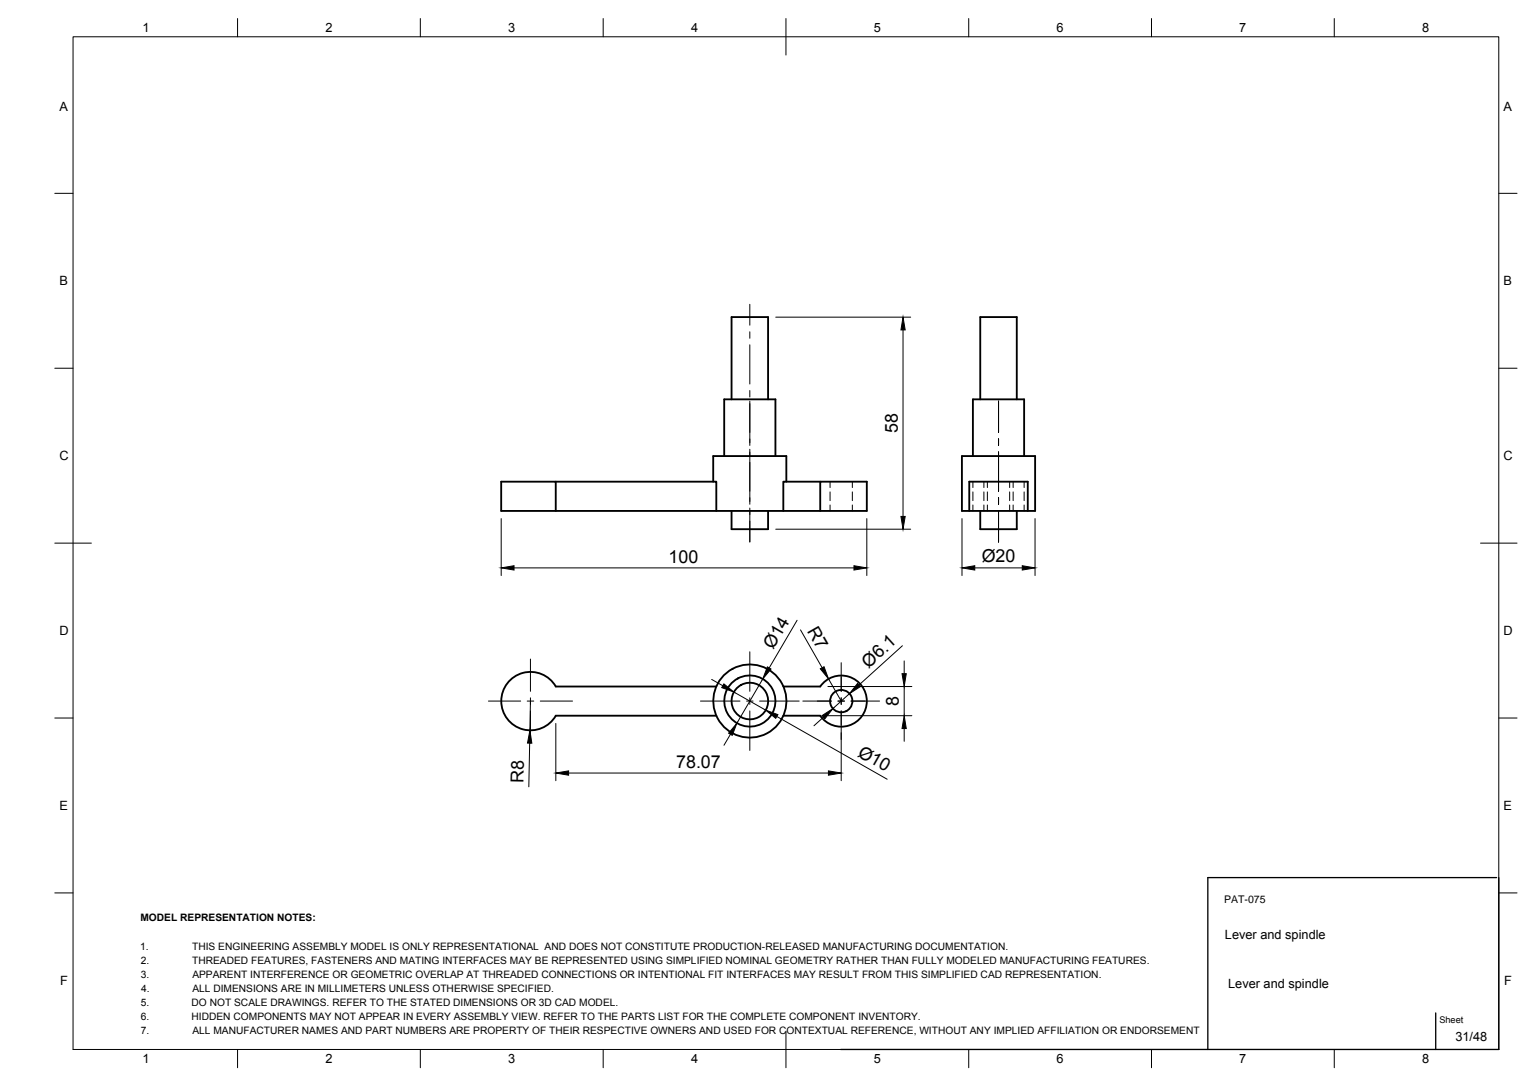
ISO-10303-21;
HEADER;
/* Generated by software containing ST-Developer
 * from STEP Tools, Inc. (www.steptools.com) 
 */

FILE_DESCRIPTION(
/* description */ ('Over-Centre Plunger Toggle Clamp on Slotted Fixture Frame'),
/* implementation_level */ '2;1');

FILE_NAME(
/* name */ 
'Lever and spindle.step',
/* time_stamp */ '2026-10-28T03:23:24-07:00',
/* author */ (''),
/* organization */ (''),
/* preprocessor_version */ 'ST-DEVELOPER v20.2',
/* originating_system */ 'Autodesk Translation Framework v15.17.0.0',
/* authorisation */ '');

FILE_SCHEMA (('AUTOMOTIVE_DESIGN { 1 0 10303 214 3 1 1 }'));
ENDSEC;

DATA;
#10=MECHANICAL_DESIGN_GEOMETRIC_PRESENTATION_REPRESENTATION('',(#545),#15212);
#453=SHAPE_REPRESENTATION_RELATIONSHIP('SRR','None',#15430,#495);
#495=ADVANCED_BREP_SHAPE_REPRESENTATION('',(#594),#15192);
#545=STYLED_ITEM('',(#15712),#594);
#594=MANIFOLD_SOLID_BREP('Body1',#8279);
#742=FACE_BOUND('',#2033,.T.);
#743=FACE_BOUND('',#2034,.T.);
#744=FACE_BOUND('',#2041,.T.);
#745=FACE_BOUND('',#2044,.T.);
#746=FACE_BOUND('',#2047,.T.);
#984=PLANE('',#9388);
#985=PLANE('',#9394);
#986=PLANE('',#9395);
#987=PLANE('',#9397);
#988=PLANE('',#9400);
#989=PLANE('',#9401);
#990=PLANE('',#9403);
#991=PLANE('',#9404);
#992=PLANE('',#9408);
#993=PLANE('',#9416);
#994=PLANE('',#9417);
#1413=FACE_OUTER_BOUND('',#2030,.T.);
#1414=FACE_OUTER_BOUND('',#2031,.T.);
#1415=FACE_OUTER_BOUND('',#2032,.T.);
#1416=FACE_OUTER_BOUND('',#2035,.T.);
#1417=FACE_OUTER_BOUND('',#2036,.T.);
#1418=FACE_OUTER_BOUND('',#2037,.T.);
#1419=FACE_OUTER_BOUND('',#2038,.T.);
#1420=FACE_OUTER_BOUND('',#2039,.T.);
#1421=FACE_OUTER_BOUND('',#2040,.T.);
#1422=FACE_OUTER_BOUND('',#2042,.T.);
#1423=FACE_OUTER_BOUND('',#2043,.T.);
#1424=FACE_OUTER_BOUND('',#2045,.T.);
#1425=FACE_OUTER_BOUND('',#2046,.T.);
#1426=FACE_OUTER_BOUND('',#2048,.T.);
#1427=FACE_OUTER_BOUND('',#2049,.T.);
#1428=FACE_OUTER_BOUND('',#2050,.T.);
#1429=FACE_OUTER_BOUND('',#2051,.T.);
#1430=FACE_OUTER_BOUND('',#2052,.T.);
#2030=EDGE_LOOP('',(#7007,#7008,#7009,#7010));
#2031=EDGE_LOOP('',(#7011,#7012,#7013,#7014));
#2032=EDGE_LOOP('',(#7015,#7016,#7017,#7018,#7019,#7020,#7021,#7022,#7023));
#2033=EDGE_LOOP('',(#7024));
#2034=EDGE_LOOP('',(#7025));
#2035=EDGE_LOOP('',(#7026,#7027,#7028,#7029));
#2036=EDGE_LOOP('',(#7030,#7031,#7032,#7033));
#2037=EDGE_LOOP('',(#7034,#7035,#7036,#7037));
#2038=EDGE_LOOP('',(#7038,#7039,#7040,#7041));
#2039=EDGE_LOOP('',(#7042,#7043,#7044,#7045));
#2040=EDGE_LOOP('',(#7046,#7047,#7048,#7049));
#2041=EDGE_LOOP('',(#7050));
#2042=EDGE_LOOP('',(#7051,#7052,#7053,#7054));
#2043=EDGE_LOOP('',(#7055));
#2044=EDGE_LOOP('',(#7056));
#2045=EDGE_LOOP('',(#7057,#7058,#7059,#7060,#7061,#7062,#7063,#7064,#7065,
#7066,#7067,#7068));
#2046=EDGE_LOOP('',(#7069));
#2047=EDGE_LOOP('',(#7070));
#2048=EDGE_LOOP('',(#7071,#7072,#7073,#7074));
#2049=EDGE_LOOP('',(#7075,#7076,#7077,#7078));
#2050=EDGE_LOOP('',(#7079,#7080,#7081,#7082));
#2051=EDGE_LOOP('',(#7083));
#2052=EDGE_LOOP('',(#7084));
#2676=LINE('',#14276,#3306);
#2677=LINE('',#14281,#3307);
#2678=LINE('',#14285,#3308);
#2679=LINE('',#14289,#3309);
#2680=LINE('',#14295,#3310);
#2681=LINE('',#14299,#3311);
#2682=LINE('',#14302,#3312);
#2683=LINE('',#14307,#3313);
#2684=LINE('',#14308,#3314);
#2685=LINE('',#14311,#3315);
#2686=LINE('',#14314,#3316);
#2687=LINE('',#14317,#3317);
#2688=LINE('',#14320,#3318);
#2689=LINE('',#14323,#3319);
#2690=LINE('',#14324,#3320);
#2691=LINE('',#14327,#3321);
#2692=LINE('',#14330,#3322);
#2693=LINE('',#14337,#3323);
#2694=LINE('',#14344,#3324);
#2695=LINE('',#14347,#3325);
#2696=LINE('',#14352,#3326);
#3306=VECTOR('',#11441,0.305);
#3307=VECTOR('',#11446,1.);
#3308=VECTOR('',#11449,1.);
#3309=VECTOR('',#11454,1.);
#3310=VECTOR('',#11459,1.);
#3311=VECTOR('',#11462,1.);
#3312=VECTOR('',#11465,1.);
#3313=VECTOR('',#11470,1.);
#3314=VECTOR('',#11471,1.);
#3315=VECTOR('',#11474,1.);
#3316=VECTOR('',#11479,1.);
#3317=VECTOR('',#11482,1.);
#3318=VECTOR('',#11485,1.);
#3319=VECTOR('',#11488,1.);
#3320=VECTOR('',#11489,1.);
#3321=VECTOR('',#11492,1.);
#3322=VECTOR('',#11497,1.);
#3323=VECTOR('',#11506,1.);
#3324=VECTOR('',#11515,0.7);
#3325=VECTOR('',#11518,0.5);
#3326=VECTOR('',#11525,0.5);
#3745=CIRCLE('',#9383,0.305);
#3746=CIRCLE('',#9384,0.305);
#3747=CIRCLE('',#9386,0.8);
#3748=CIRCLE('',#9387,0.8);
#3749=CIRCLE('',#9389,1.);
#3750=CIRCLE('',#9390,1.);
#3751=CIRCLE('',#9391,0.7);
#3752=CIRCLE('',#9392,1.);
#3753=CIRCLE('',#9393,0.5);
#3754=CIRCLE('',#9396,1.);
#3755=CIRCLE('',#9399,0.7);
#3756=CIRCLE('',#9402,1.);
#3757=CIRCLE('',#9405,1.);
#3758=CIRCLE('',#9406,0.7);
#3759=CIRCLE('',#9409,0.7);
#3760=CIRCLE('',#9410,0.5);
#3761=CIRCLE('',#9413,0.5);
#3762=CIRCLE('',#9415,0.5);
#4345=VERTEX_POINT('',#14273);
#4346=VERTEX_POINT('',#14275);
#4347=VERTEX_POINT('',#14279);
#4348=VERTEX_POINT('',#14280);
#4349=VERTEX_POINT('',#14282);
#4350=VERTEX_POINT('',#14284);
#4351=VERTEX_POINT('',#14288);
#4352=VERTEX_POINT('',#14290);
#4353=VERTEX_POINT('',#14292);
#4354=VERTEX_POINT('',#14294);
#4355=VERTEX_POINT('',#14296);
#4356=VERTEX_POINT('',#14298);
#4357=VERTEX_POINT('',#14300);
#4358=VERTEX_POINT('',#14303);
#4359=VERTEX_POINT('',#14306);
#4360=VERTEX_POINT('',#14310);
#4361=VERTEX_POINT('',#14316);
#4362=VERTEX_POINT('',#14318);
#4363=VERTEX_POINT('',#14322);
#4364=VERTEX_POINT('',#14326);
#4365=VERTEX_POINT('',#14332);
#4366=VERTEX_POINT('',#14334);
#4367=VERTEX_POINT('',#14339);
#4368=VERTEX_POINT('',#14341);
#4369=VERTEX_POINT('',#14346);
#4370=VERTEX_POINT('',#14350);
#5264=EDGE_CURVE('',#4345,#4345,#3745,.T.);
#5265=EDGE_CURVE('',#4345,#4346,#2676,.T.);
#5266=EDGE_CURVE('',#4346,#4346,#3746,.T.);
#5267=EDGE_CURVE('',#4347,#4348,#2677,.T.);
#5268=EDGE_CURVE('',#4349,#4347,#3747,.T.);
#5269=EDGE_CURVE('',#4350,#4349,#2678,.T.);
#5270=EDGE_CURVE('',#4350,#4348,#3748,.T.);
#5271=EDGE_CURVE('',#4351,#4350,#2679,.T.);
#5272=EDGE_CURVE('',#4352,#4351,#3749,.T.);
#5273=EDGE_CURVE('',#4353,#4352,#3750,.T.);
#5274=EDGE_CURVE('',#4354,#4353,#2680,.T.);
#5275=EDGE_CURVE('',#4355,#4354,#3751,.T.);
#5276=EDGE_CURVE('',#4356,#4355,#2681,.T.);
#5277=EDGE_CURVE('',#4357,#4356,#3752,.T.);
#5278=EDGE_CURVE('',#4348,#4357,#2682,.T.);
#5279=EDGE_CURVE('',#4358,#4358,#3753,.T.);
#5280=EDGE_CURVE('',#4359,#4349,#2683,.T.);
#5281=EDGE_CURVE('',#4351,#4359,#2684,.T.);
#5282=EDGE_CURVE('',#4347,#4360,#2685,.T.);
#5283=EDGE_CURVE('',#4359,#4360,#3754,.T.);
#5284=EDGE_CURVE('',#4360,#4357,#2686,.T.);
#5285=EDGE_CURVE('',#4361,#4354,#2687,.T.);
#5286=EDGE_CURVE('',#4362,#4361,#3755,.T.);
#5287=EDGE_CURVE('',#4355,#4362,#2688,.T.);
#5288=EDGE_CURVE('',#4363,#4362,#2689,.T.);
#5289=EDGE_CURVE('',#4356,#4363,#2690,.T.);
#5290=EDGE_CURVE('',#4361,#4364,#2691,.T.);
#5291=EDGE_CURVE('',#4363,#4364,#3756,.T.);
#5292=EDGE_CURVE('',#4364,#4353,#2692,.T.);
#5293=EDGE_CURVE('',#4365,#4365,#3757,.T.);
#5294=EDGE_CURVE('',#4366,#4366,#3758,.T.);
#5295=EDGE_CURVE('',#4365,#4352,#2693,.T.);
#5296=EDGE_CURVE('',#4367,#4367,#3759,.T.);
#5297=EDGE_CURVE('',#4368,#4368,#3760,.T.);
#5298=EDGE_CURVE('',#4367,#4366,#2694,.T.);
#5299=EDGE_CURVE('',#4358,#4369,#2695,.T.);
#5300=EDGE_CURVE('',#4369,#4369,#3761,.T.);
#5301=EDGE_CURVE('',#4370,#4370,#3762,.T.);
#5302=EDGE_CURVE('',#4370,#4368,#2696,.T.);
#7007=ORIENTED_EDGE('',*,*,#5264,.F.);
#7008=ORIENTED_EDGE('',*,*,#5265,.T.);
#7009=ORIENTED_EDGE('',*,*,#5266,.F.);
#7010=ORIENTED_EDGE('',*,*,#5265,.F.);
#7011=ORIENTED_EDGE('',*,*,#5267,.F.);
#7012=ORIENTED_EDGE('',*,*,#5268,.F.);
#7013=ORIENTED_EDGE('',*,*,#5269,.F.);
#7014=ORIENTED_EDGE('',*,*,#5270,.T.);
#7015=ORIENTED_EDGE('',*,*,#5270,.F.);
#7016=ORIENTED_EDGE('',*,*,#5271,.F.);
#7017=ORIENTED_EDGE('',*,*,#5272,.F.);
#7018=ORIENTED_EDGE('',*,*,#5273,.F.);
#7019=ORIENTED_EDGE('',*,*,#5274,.F.);
#7020=ORIENTED_EDGE('',*,*,#5275,.F.);
#7021=ORIENTED_EDGE('',*,*,#5276,.F.);
#7022=ORIENTED_EDGE('',*,*,#5277,.F.);
#7023=ORIENTED_EDGE('',*,*,#5278,.F.);
#7024=ORIENTED_EDGE('',*,*,#5264,.T.);
#7025=ORIENTED_EDGE('',*,*,#5279,.F.);
#7026=ORIENTED_EDGE('',*,*,#5269,.T.);
#7027=ORIENTED_EDGE('',*,*,#5280,.F.);
#7028=ORIENTED_EDGE('',*,*,#5281,.F.);
#7029=ORIENTED_EDGE('',*,*,#5271,.T.);
#7030=ORIENTED_EDGE('',*,*,#5282,.T.);
#7031=ORIENTED_EDGE('',*,*,#5283,.F.);
#7032=ORIENTED_EDGE('',*,*,#5280,.T.);
#7033=ORIENTED_EDGE('',*,*,#5268,.T.);
#7034=ORIENTED_EDGE('',*,*,#5267,.T.);
#7035=ORIENTED_EDGE('',*,*,#5278,.T.);
#7036=ORIENTED_EDGE('',*,*,#5284,.F.);
#7037=ORIENTED_EDGE('',*,*,#5282,.F.);
#7038=ORIENTED_EDGE('',*,*,#5285,.F.);
#7039=ORIENTED_EDGE('',*,*,#5286,.F.);
#7040=ORIENTED_EDGE('',*,*,#5287,.F.);
#7041=ORIENTED_EDGE('',*,*,#5275,.T.);
#7042=ORIENTED_EDGE('',*,*,#5287,.T.);
#7043=ORIENTED_EDGE('',*,*,#5288,.F.);
#7044=ORIENTED_EDGE('',*,*,#5289,.F.);
#7045=ORIENTED_EDGE('',*,*,#5276,.T.);
#7046=ORIENTED_EDGE('',*,*,#5290,.T.);
#7047=ORIENTED_EDGE('',*,*,#5291,.F.);
#7048=ORIENTED_EDGE('',*,*,#5288,.T.);
#7049=ORIENTED_EDGE('',*,*,#5286,.T.);
#7050=ORIENTED_EDGE('',*,*,#5266,.T.);
#7051=ORIENTED_EDGE('',*,*,#5285,.T.);
#7052=ORIENTED_EDGE('',*,*,#5274,.T.);
#7053=ORIENTED_EDGE('',*,*,#5292,.F.);
#7054=ORIENTED_EDGE('',*,*,#5290,.F.);
#7055=ORIENTED_EDGE('',*,*,#5293,.T.);
#7056=ORIENTED_EDGE('',*,*,#5294,.F.);
#7057=ORIENTED_EDGE('',*,*,#5293,.F.);
#7058=ORIENTED_EDGE('',*,*,#5295,.T.);
#7059=ORIENTED_EDGE('',*,*,#5272,.T.);
#7060=ORIENTED_EDGE('',*,*,#5281,.T.);
#7061=ORIENTED_EDGE('',*,*,#5283,.T.);
#7062=ORIENTED_EDGE('',*,*,#5284,.T.);
#7063=ORIENTED_EDGE('',*,*,#5277,.T.);
#7064=ORIENTED_EDGE('',*,*,#5289,.T.);
#7065=ORIENTED_EDGE('',*,*,#5291,.T.);
#7066=ORIENTED_EDGE('',*,*,#5292,.T.);
#7067=ORIENTED_EDGE('',*,*,#5273,.T.);
#7068=ORIENTED_EDGE('',*,*,#5295,.F.);
#7069=ORIENTED_EDGE('',*,*,#5296,.T.);
#7070=ORIENTED_EDGE('',*,*,#5297,.F.);
#7071=ORIENTED_EDGE('',*,*,#5296,.F.);
#7072=ORIENTED_EDGE('',*,*,#5298,.T.);
#7073=ORIENTED_EDGE('',*,*,#5294,.T.);
#7074=ORIENTED_EDGE('',*,*,#5298,.F.);
#7075=ORIENTED_EDGE('',*,*,#5279,.T.);
#7076=ORIENTED_EDGE('',*,*,#5299,.T.);
#7077=ORIENTED_EDGE('',*,*,#5300,.T.);
#7078=ORIENTED_EDGE('',*,*,#5299,.F.);
#7079=ORIENTED_EDGE('',*,*,#5301,.F.);
#7080=ORIENTED_EDGE('',*,*,#5302,.T.);
#7081=ORIENTED_EDGE('',*,*,#5297,.T.);
#7082=ORIENTED_EDGE('',*,*,#5302,.F.);
#7083=ORIENTED_EDGE('',*,*,#5301,.T.);
#7084=ORIENTED_EDGE('',*,*,#5300,.F.);
#7712=CYLINDRICAL_SURFACE('',#9382,0.305);
#7713=CYLINDRICAL_SURFACE('',#9385,0.8);
#7714=CYLINDRICAL_SURFACE('',#9398,0.7);
#7715=CYLINDRICAL_SURFACE('',#9407,1.);
#7716=CYLINDRICAL_SURFACE('',#9411,0.7);
#7717=CYLINDRICAL_SURFACE('',#9412,0.5);
#7718=CYLINDRICAL_SURFACE('',#9414,0.5);
#8085=ADVANCED_FACE('',(#1413),#7712,.F.);
#8086=ADVANCED_FACE('',(#1414),#7713,.T.);
#8087=ADVANCED_FACE('',(#1415,#742,#743),#984,.F.);
#8088=ADVANCED_FACE('',(#1416),#985,.T.);
#8089=ADVANCED_FACE('',(#1417),#986,.T.);
#8090=ADVANCED_FACE('',(#1418),#987,.T.);
#8091=ADVANCED_FACE('',(#1419),#7714,.T.);
#8092=ADVANCED_FACE('',(#1420),#988,.T.);
#8093=ADVANCED_FACE('',(#1421,#744),#989,.T.);
#8094=ADVANCED_FACE('',(#1422),#990,.T.);
#8095=ADVANCED_FACE('',(#1423,#745),#991,.T.);
#8096=ADVANCED_FACE('',(#1424),#7715,.T.);
#8097=ADVANCED_FACE('',(#1425,#746),#992,.T.);
#8098=ADVANCED_FACE('',(#1426),#7716,.T.);
#8099=ADVANCED_FACE('',(#1427),#7717,.T.);
#8100=ADVANCED_FACE('',(#1428),#7718,.T.);
#8101=ADVANCED_FACE('',(#1429),#993,.T.);
#8102=ADVANCED_FACE('',(#1430),#994,.F.);
#8279=CLOSED_SHELL('',(#8085,#8086,#8087,#8088,#8089,#8090,#8091,#8092,
#8093,#8094,#8095,#8096,#8097,#8098,#8099,#8100,#8101,#8102));
#9381=AXIS2_PLACEMENT_3D('',#14271,#11435,#11436);
#9382=AXIS2_PLACEMENT_3D('',#14272,#11437,#11438);
#9383=AXIS2_PLACEMENT_3D('',#14274,#11439,#11440);
#9384=AXIS2_PLACEMENT_3D('',#14277,#11442,#11443);
#9385=AXIS2_PLACEMENT_3D('',#14278,#11444,#11445);
#9386=AXIS2_PLACEMENT_3D('',#14283,#11447,#11448);
#9387=AXIS2_PLACEMENT_3D('',#14286,#11450,#11451);
#9388=AXIS2_PLACEMENT_3D('',#14287,#11452,#11453);
#9389=AXIS2_PLACEMENT_3D('',#14291,#11455,#11456);
#9390=AXIS2_PLACEMENT_3D('',#14293,#11457,#11458);
#9391=AXIS2_PLACEMENT_3D('',#14297,#11460,#11461);
#9392=AXIS2_PLACEMENT_3D('',#14301,#11463,#11464);
#9393=AXIS2_PLACEMENT_3D('',#14304,#11466,#11467);
#9394=AXIS2_PLACEMENT_3D('',#14305,#11468,#11469);
#9395=AXIS2_PLACEMENT_3D('',#14309,#11472,#11473);
#9396=AXIS2_PLACEMENT_3D('',#14312,#11475,#11476);
#9397=AXIS2_PLACEMENT_3D('',#14313,#11477,#11478);
#9398=AXIS2_PLACEMENT_3D('',#14315,#11480,#11481);
#9399=AXIS2_PLACEMENT_3D('',#14319,#11483,#11484);
#9400=AXIS2_PLACEMENT_3D('',#14321,#11486,#11487);
#9401=AXIS2_PLACEMENT_3D('',#14325,#11490,#11491);
#9402=AXIS2_PLACEMENT_3D('',#14328,#11493,#11494);
#9403=AXIS2_PLACEMENT_3D('',#14329,#11495,#11496);
#9404=AXIS2_PLACEMENT_3D('',#14331,#11498,#11499);
#9405=AXIS2_PLACEMENT_3D('',#14333,#11500,#11501);
#9406=AXIS2_PLACEMENT_3D('',#14335,#11502,#11503);
#9407=AXIS2_PLACEMENT_3D('',#14336,#11504,#11505);
#9408=AXIS2_PLACEMENT_3D('',#14338,#11507,#11508);
#9409=AXIS2_PLACEMENT_3D('',#14340,#11509,#11510);
#9410=AXIS2_PLACEMENT_3D('',#14342,#11511,#11512);
#9411=AXIS2_PLACEMENT_3D('',#14343,#11513,#11514);
#9412=AXIS2_PLACEMENT_3D('',#14345,#11516,#11517);
#9413=AXIS2_PLACEMENT_3D('',#14348,#11519,#11520);
#9414=AXIS2_PLACEMENT_3D('',#14349,#11521,#11522);
#9415=AXIS2_PLACEMENT_3D('',#14351,#11523,#11524);
#9416=AXIS2_PLACEMENT_3D('',#14353,#11526,#11527);
#9417=AXIS2_PLACEMENT_3D('',#14354,#11528,#11529);
#11435=DIRECTION('axis',(0.,0.,1.));
#11436=DIRECTION('refdir',(1.,0.,0.));
#11437=DIRECTION('center_axis',(0.,1.,0.));
#11438=DIRECTION('ref_axis',(1.,0.,0.));
#11439=DIRECTION('center_axis',(0.,1.,0.));
#11440=DIRECTION('ref_axis',(1.,0.,0.));
#11441=DIRECTION('',(0.,1.,0.));
#11442=DIRECTION('center_axis',(0.,-1.,0.));
#11443=DIRECTION('ref_axis',(1.,0.,0.));
#11444=DIRECTION('center_axis',(0.,1.,0.));
#11445=DIRECTION('ref_axis',(-0.46947156278589,0.,0.882947592858928));
#11446=DIRECTION('',(0.,-1.,0.));
#11447=DIRECTION('center_axis',(0.,1.,0.));
#11448=DIRECTION('ref_axis',(1.,0.,0.));
#11449=DIRECTION('',(0.,1.,0.));
#11450=DIRECTION('center_axis',(0.,1.,0.));
#11451=DIRECTION('ref_axis',(1.,0.,0.));
#11452=DIRECTION('center_axis',(0.,1.,0.));
#11453=DIRECTION('ref_axis',(1.,0.,0.));
#11454=DIRECTION('',(-0.469471562785891,0.,0.882947592858927));
#11455=DIRECTION('center_axis',(0.,1.,0.));
#11456=DIRECTION('ref_axis',(1.,0.,0.));
#11457=DIRECTION('center_axis',(0.,1.,0.));
#11458=DIRECTION('ref_axis',(1.,0.,0.));
#11459=DIRECTION('',(-0.469471562785891,0.,0.882947592858927));
#11460=DIRECTION('center_axis',(0.,1.,0.));
#11461=DIRECTION('ref_axis',(1.,0.,0.));
#11462=DIRECTION('',(0.469471562785891,0.,-0.882947592858927));
#11463=DIRECTION('center_axis',(0.,1.,0.));
#11464=DIRECTION('ref_axis',(1.,0.,0.));
#11465=DIRECTION('',(0.469471562785891,0.,-0.882947592858927));
#11466=DIRECTION('center_axis',(0.,-1.,0.));
#11467=DIRECTION('ref_axis',(1.,0.,0.));
#11468=DIRECTION('center_axis',(-0.882947592858927,0.,-0.469471562785891));
#11469=DIRECTION('ref_axis',(-0.469471562785891,0.,0.882947592858927));
#11470=DIRECTION('',(-0.469471562785891,0.,0.882947592858927));
#11471=DIRECTION('',(0.,1.,0.));
#11472=DIRECTION('center_axis',(0.,1.,0.));
#11473=DIRECTION('ref_axis',(0.,0.,1.));
#11474=DIRECTION('',(0.469471562785891,0.,-0.882947592858927));
#11475=DIRECTION('center_axis',(0.,1.,0.));
#11476=DIRECTION('ref_axis',(1.,0.,0.));
#11477=DIRECTION('center_axis',(0.882947592858927,0.,0.469471562785891));
#11478=DIRECTION('ref_axis',(0.469471562785891,0.,-0.882947592858927));
#11479=DIRECTION('',(0.,-1.,0.));
#11480=DIRECTION('center_axis',(0.,1.,0.));
#11481=DIRECTION('ref_axis',(0.46947156278589,0.,-0.882947592858927));
#11482=DIRECTION('',(0.,-1.,0.));
#11483=DIRECTION('center_axis',(0.,1.,0.));
#11484=DIRECTION('ref_axis',(1.,0.,0.));
#11485=DIRECTION('',(0.,1.,0.));
#11486=DIRECTION('center_axis',(0.882947592858927,0.,0.469471562785891));
#11487=DIRECTION('ref_axis',(0.469471562785891,0.,-0.882947592858927));
#11488=DIRECTION('',(0.469471562785891,0.,-0.882947592858927));
#11489=DIRECTION('',(0.,1.,0.));
#11490=DIRECTION('center_axis',(0.,1.,0.));
#11491=DIRECTION('ref_axis',(0.,0.,1.));
#11492=DIRECTION('',(-0.469471562785891,0.,0.882947592858927));
#11493=DIRECTION('center_axis',(0.,1.,0.));
#11494=DIRECTION('ref_axis',(1.,0.,0.));
#11495=DIRECTION('center_axis',(-0.882947592858927,0.,-0.469471562785891));
#11496=DIRECTION('ref_axis',(-0.469471562785891,0.,0.882947592858927));
#11497=DIRECTION('',(0.,-1.,0.));
#11498=DIRECTION('center_axis',(0.,1.,0.));
#11499=DIRECTION('ref_axis',(1.,0.,0.));
#11500=DIRECTION('center_axis',(0.,1.,0.));
#11501=DIRECTION('ref_axis',(1.,0.,0.));
#11502=DIRECTION('center_axis',(0.,1.,0.));
#11503=DIRECTION('ref_axis',(1.,0.,0.));
#11504=DIRECTION('center_axis',(0.,1.,0.));
#11505=DIRECTION('ref_axis',(1.,0.,0.));
#11506=DIRECTION('',(0.,-1.,0.));
#11507=DIRECTION('center_axis',(0.,1.,0.));
#11508=DIRECTION('ref_axis',(1.,0.,0.));
#11509=DIRECTION('center_axis',(0.,1.,0.));
#11510=DIRECTION('ref_axis',(1.,0.,0.));
#11511=DIRECTION('center_axis',(0.,1.,0.));
#11512=DIRECTION('ref_axis',(1.,0.,0.));
#11513=DIRECTION('center_axis',(0.,1.,0.));
#11514=DIRECTION('ref_axis',(1.,0.,0.));
#11515=DIRECTION('',(0.,-1.,0.));
#11516=DIRECTION('center_axis',(0.,1.,0.));
#11517=DIRECTION('ref_axis',(1.,0.,0.));
#11518=DIRECTION('',(0.,-1.,0.));
#11519=DIRECTION('center_axis',(0.,1.,0.));
#11520=DIRECTION('ref_axis',(1.,0.,0.));
#11521=DIRECTION('center_axis',(0.,1.,0.));
#11522=DIRECTION('ref_axis',(1.,0.,0.));
#11523=DIRECTION('center_axis',(0.,1.,0.));
#11524=DIRECTION('ref_axis',(1.,0.,0.));
#11525=DIRECTION('',(0.,-1.,0.));
#11526=DIRECTION('center_axis',(0.,1.,0.));
#11527=DIRECTION('ref_axis',(1.,0.,0.));
#11528=DIRECTION('center_axis',(0.,1.,0.));
#11529=DIRECTION('ref_axis',(1.,0.,0.));
#14271=CARTESIAN_POINT('',(0.,0.,0.));
#14272=CARTESIAN_POINT('Origin',(-2.82632109303527,-3.6,8.79263101785268));
#14273=CARTESIAN_POINT('',(-3.13132109303527,-3.5,8.79263101785268));
#14274=CARTESIAN_POINT('Origin',(-2.82632109303527,-3.5,8.79263101785268));
#14275=CARTESIAN_POINT('',(-3.13132109303527,-2.7,8.79263101785268));
#14276=CARTESIAN_POINT('',(-3.13132109303527,-3.6,8.79263101785268));
#14277=CARTESIAN_POINT('Origin',(-2.82632109303527,-2.7,8.79263101785268));
#14278=CARTESIAN_POINT('Origin',(-6.81682937671534,-3.5,16.2976855571536));
#14279=CARTESIAN_POINT('',(-6.1383908997902,-2.7,15.873750145767));
#14280=CARTESIAN_POINT('',(-6.1383908997902,-3.5,15.873750145767));
#14281=CARTESIAN_POINT('',(-6.1383908997902,-3.5,15.873750145767));
#14282=CARTESIAN_POINT('',(-6.84474897407734,-2.7,15.4981728955383));
#14283=CARTESIAN_POINT('Origin',(-6.81682937671534,-2.7,16.2976855571536));
#14284=CARTESIAN_POINT('',(-6.84474897407734,-3.5,15.4981728955383));
#14285=CARTESIAN_POINT('',(-6.84474897407734,-3.5,15.4981728955383));
#14286=CARTESIAN_POINT('Origin',(-6.81682937671534,-3.5,16.2976855571536));
#14287=CARTESIAN_POINT('Origin',(-4.,-3.5,11.));
#14288=CARTESIAN_POINT('',(-4.78345683176268,-3.5,11.6214462106767));
#14289=CARTESIAN_POINT('',(-4.35317903714357,-3.5,10.8122113748856));
#14290=CARTESIAN_POINT('',(-5.,-3.5,11.));
#14291=CARTESIAN_POINT('Origin',(-4.,-3.5,11.));
#14292=CARTESIAN_POINT('',(-3.92290124252446,-3.5,10.0029765390946));
#14293=CARTESIAN_POINT('Origin',(-4.,-3.5,11.));
#14294=CARTESIAN_POINT('',(-3.44919101049801,-3.5,9.11205716881713));
#14295=CARTESIAN_POINT('',(-3.17950013017884,-3.5,8.60484239273833));
#14296=CARTESIAN_POINT('',(-2.74283293621087,-3.5,9.48763441904585));
#14297=CARTESIAN_POINT('Origin',(-2.82632109303527,-3.5,8.79263101785268));
#14298=CARTESIAN_POINT('',(-3.21654316823732,-3.5,10.3785537893233));
#14299=CARTESIAN_POINT('',(-3.64682096285643,-3.5,11.1877886251144));
#14300=CARTESIAN_POINT('',(-4.07709875747554,-3.5,11.9970234609054));
#14301=CARTESIAN_POINT('Origin',(-4.,-3.5,11.));
#14302=CARTESIAN_POINT('',(-6.46365033957177,-3.5,16.4854741822679));
#14303=CARTESIAN_POINT('',(-4.5,-3.5,11.));
#14304=CARTESIAN_POINT('Origin',(-4.,-3.5,11.));
#14305=CARTESIAN_POINT('Origin',(-4.35317903714357,-3.5,10.8122113748856));
#14306=CARTESIAN_POINT('',(-4.78345683176268,-2.7,11.6214462106767));
#14307=CARTESIAN_POINT('',(-4.35317903714357,-2.7,10.8122113748856));
#14308=CARTESIAN_POINT('',(-4.78345683176268,-3.5,11.6214462106767));
#14309=CARTESIAN_POINT('Origin',(-5.40841468835767,-2.7,13.6488427785768));
#14310=CARTESIAN_POINT('',(-4.07709875747554,-2.7,11.9970234609054));
#14311=CARTESIAN_POINT('',(-6.46365033957177,-2.7,16.4854741822679));
#14312=CARTESIAN_POINT('Origin',(-4.,-2.7,11.));
#14313=CARTESIAN_POINT('Origin',(-6.46365033957177,-3.5,16.4854741822679));
#14314=CARTESIAN_POINT('',(-4.07709875747554,-3.5,11.9970234609054));
#14315=CARTESIAN_POINT('Origin',(-2.82632109303527,-3.5,8.79263101785268));
#14316=CARTESIAN_POINT('',(-3.44919101049801,-2.7,9.11205716881713));
#14317=CARTESIAN_POINT('',(-3.44919101049801,-3.5,9.11205716881713));
#14318=CARTESIAN_POINT('',(-2.74283293621087,-2.7,9.48763441904585));
#14319=CARTESIAN_POINT('Origin',(-2.82632109303527,-2.7,8.79263101785268));
#14320=CARTESIAN_POINT('',(-2.74283293621087,-3.5,9.48763441904585));
#14321=CARTESIAN_POINT('Origin',(-3.64682096285643,-3.5,11.1877886251144));
#14322=CARTESIAN_POINT('',(-3.21654316823732,-2.7,10.3785537893233));
#14323=CARTESIAN_POINT('',(-3.64682096285643,-2.7,11.1877886251144));
#14324=CARTESIAN_POINT('',(-3.21654316823732,-3.5,10.3785537893233));
#14325=CARTESIAN_POINT('Origin',(-3.41316054651764,-2.7,9.89631550892634));
#14326=CARTESIAN_POINT('',(-3.92290124252446,-2.7,10.0029765390946));
#14327=CARTESIAN_POINT('',(-3.17950013017884,-2.7,8.60484239273833));
#14328=CARTESIAN_POINT('Origin',(-4.,-2.7,11.));
#14329=CARTESIAN_POINT('Origin',(-3.17950013017884,-3.5,8.60484239273833));
#14330=CARTESIAN_POINT('',(-3.92290124252446,-3.5,10.0029765390946));
#14331=CARTESIAN_POINT('Origin',(-4.,-2.,11.));
#14332=CARTESIAN_POINT('',(-5.,-2.,11.));
#14333=CARTESIAN_POINT('Origin',(-4.,-2.,11.));
#14334=CARTESIAN_POINT('',(-4.7,-2.,11.));
#14335=CARTESIAN_POINT('Origin',(-4.,-2.,11.));
#14336=CARTESIAN_POINT('Origin',(-4.,-3.5,11.));
#14337=CARTESIAN_POINT('',(-5.,-3.5,11.));
#14338=CARTESIAN_POINT('Origin',(-4.,-0.45,11.));
#14339=CARTESIAN_POINT('',(-4.7,-0.45,11.));
#14340=CARTESIAN_POINT('Origin',(-4.,-0.45,11.));
#14341=CARTESIAN_POINT('',(-4.5,-0.45,11.));
#14342=CARTESIAN_POINT('Origin',(-4.,-0.45,11.));
#14343=CARTESIAN_POINT('Origin',(-4.,-2.,11.));
#14344=CARTESIAN_POINT('',(-4.7,-2.,11.));
#14345=CARTESIAN_POINT('Origin',(-4.,-4.,11.));
#14346=CARTESIAN_POINT('',(-4.5,-4.,11.));
#14347=CARTESIAN_POINT('',(-4.5,-4.,11.));
#14348=CARTESIAN_POINT('Origin',(-4.,-4.,11.));
#14349=CARTESIAN_POINT('Origin',(-4.,-4.,11.));
#14350=CARTESIAN_POINT('',(-4.5,1.8,11.));
#14351=CARTESIAN_POINT('Origin',(-4.,1.8,11.));
#14352=CARTESIAN_POINT('',(-4.5,-4.,11.));
#14353=CARTESIAN_POINT('Origin',(-4.,1.8,11.));
#14354=CARTESIAN_POINT('Origin',(-4.,-4.,11.));
#15142=UNCERTAINTY_MEASURE_WITH_UNIT(LENGTH_MEASURE(0.001),#15213,
'DISTANCE_ACCURACY_VALUE',
'Maximum model space distance between geometric entities at asserted c
onnectivities');
#15162=UNCERTAINTY_MEASURE_WITH_UNIT(LENGTH_MEASURE(0.001),#15213,
'DISTANCE_ACCURACY_VALUE',
'Maximum model space distance between geometric entities at asserted c
onnectivities');
#15192=(
GEOMETRIC_REPRESENTATION_CONTEXT(3)
GLOBAL_UNCERTAINTY_ASSIGNED_CONTEXT((#15142))
GLOBAL_UNIT_ASSIGNED_CONTEXT((#15213,#15215,#15216))
REPRESENTATION_CONTEXT('','3D')
);
#15212=(
GEOMETRIC_REPRESENTATION_CONTEXT(3)
GLOBAL_UNCERTAINTY_ASSIGNED_CONTEXT((#15162))
GLOBAL_UNIT_ASSIGNED_CONTEXT((#15213,#15215,#15216))
REPRESENTATION_CONTEXT('','3D')
);
#15213=(
LENGTH_UNIT()
NAMED_UNIT(*)
SI_UNIT(.CENTI.,.METRE.)
);
#15215=(
NAMED_UNIT(*)
PLANE_ANGLE_UNIT()
SI_UNIT($,.RADIAN.)
);
#15216=(
NAMED_UNIT(*)
SI_UNIT($,.STERADIAN.)
SOLID_ANGLE_UNIT()
);
#15246=SHAPE_DEFINITION_REPRESENTATION(#15302,#15430);
#15302=PRODUCT_DEFINITION_SHAPE('',$,#15480);
#15430=SHAPE_REPRESENTATION('',(#9381),#15192);
#15450=PRODUCT_DEFINITION_CONTEXT('part definition',#15599,'design');
#15480=PRODUCT_DEFINITION('Lever and spindle','Lever and spindle',#15529,
#15450);
#15529=PRODUCT_DEFINITION_FORMATION('',$,#15630);
#15599=APPLICATION_CONTEXT(
'Core Data for Automotive Mechanical Design Process');
#15600=PRODUCT_CONTEXT('part definition',#15599,'mechanical');
#15630=PRODUCT('Lever and spindle','Lever and spindle',
'Lever and spindle',(#15600));
#15706=COLOUR_RGB('Sky Blue',0.24,0.69,0.87);
#15707=FILL_AREA_STYLE_COLOUR('',#15706);
#15708=FILL_AREA_STYLE('',(#15707));
#15709=SURFACE_STYLE_FILL_AREA(#15708);
#15710=SURFACE_SIDE_STYLE('',(#15709));
#15711=SURFACE_STYLE_USAGE(.BOTH.,#15710);
#15712=PRESENTATION_STYLE_ASSIGNMENT((#15711));
ENDSEC;
END-ISO-10303-21;
